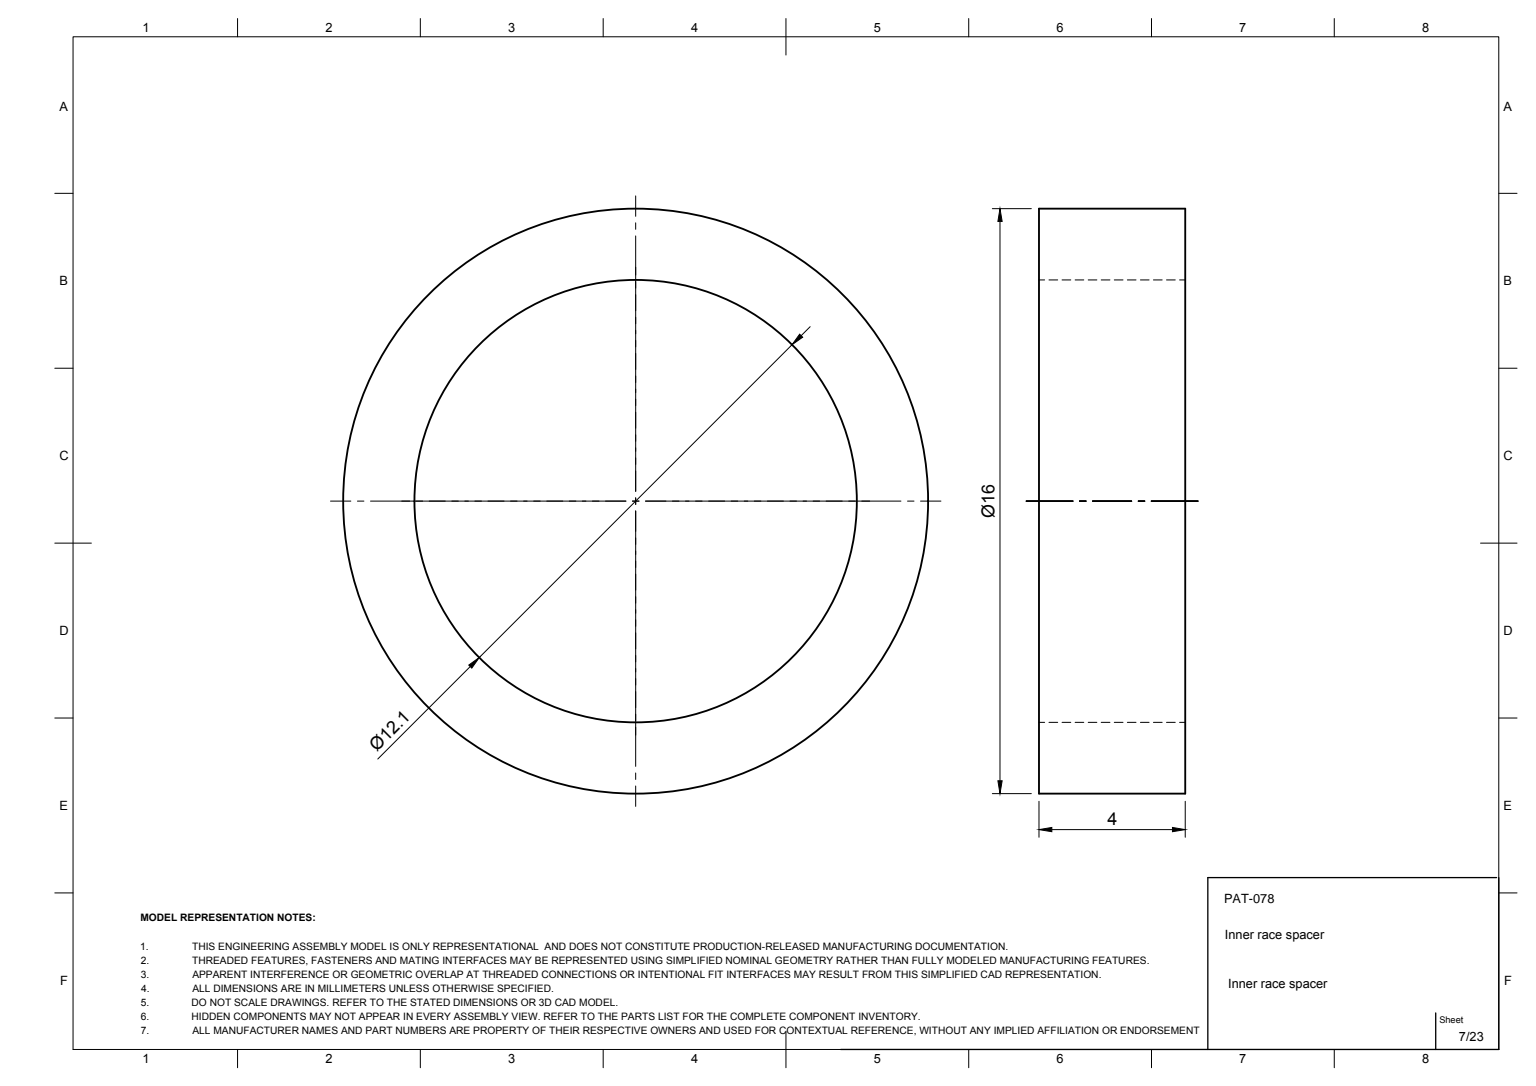
ISO-10303-21;
HEADER;
/* Generated by software containing ST-Developer
 * from STEP Tools, Inc. (www.steptools.com) 
 */

FILE_DESCRIPTION(
/* description */ ('Pedal-braked fixed caster'),
/* implementation_level */ '2;1');

FILE_NAME(
/* name */ 'Inner race spacer.step',
/* time_stamp */ '2026-10-28T03:26:52-07:00',
/* author */ (''),
/* organization */ (''),
/* preprocessor_version */ 'ST-DEVELOPER v20.2',
/* originating_system */ 'Autodesk Translation Framework v15.17.0.0',
/* authorisation */ '');

FILE_SCHEMA (('AUTOMOTIVE_DESIGN { 1 0 10303 214 3 1 1 }'));
ENDSEC;

DATA;
#10=MECHANICAL_DESIGN_GEOMETRIC_PRESENTATION_REPRESENTATION('',(#208),#5734);
#174=SHAPE_REPRESENTATION_RELATIONSHIP('SRR','None',#5812,#191);
#191=ADVANCED_BREP_SHAPE_REPRESENTATION('',(#232),#5716);
#208=STYLED_ITEM('',(#5984),#232);
#232=MANIFOLD_SOLID_BREP('Body1',#2989);
#264=CYLINDRICAL_SURFACE('',#3276,0.605);
#265=CYLINDRICAL_SURFACE('',#3279,0.8);
#313=FACE_BOUND('',#724,.T.);
#314=FACE_BOUND('',#726,.T.);
#362=CIRCLE('',#3277,0.605);
#363=CIRCLE('',#3278,0.605);
#364=CIRCLE('',#3280,0.8);
#365=CIRCLE('',#3281,0.8);
#525=FACE_OUTER_BOUND('',#721,.T.);
#526=FACE_OUTER_BOUND('',#722,.T.);
#527=FACE_OUTER_BOUND('',#723,.T.);
#528=FACE_OUTER_BOUND('',#725,.T.);
#721=EDGE_LOOP('',(#2186,#2187,#2188,#2189));
#722=EDGE_LOOP('',(#2190,#2191,#2192,#2193));
#723=EDGE_LOOP('',(#2194));
#724=EDGE_LOOP('',(#2195));
#725=EDGE_LOOP('',(#2196));
#726=EDGE_LOOP('',(#2197));
#978=LINE('',#4758,#1190);
#979=LINE('',#4764,#1191);
#1190=VECTOR('',#3818,0.605);
#1191=VECTOR('',#3825,0.8);
#1383=VERTEX_POINT('',#4755);
#1384=VERTEX_POINT('',#4757);
#1385=VERTEX_POINT('',#4761);
#1386=VERTEX_POINT('',#4763);
#1683=EDGE_CURVE('',#1383,#1383,#362,.T.);
#1684=EDGE_CURVE('',#1383,#1384,#978,.T.);
#1685=EDGE_CURVE('',#1384,#1384,#363,.T.);
#1686=EDGE_CURVE('',#1385,#1385,#364,.T.);
#1687=EDGE_CURVE('',#1385,#1386,#979,.T.);
#1688=EDGE_CURVE('',#1386,#1386,#365,.T.);
#2186=ORIENTED_EDGE('',*,*,#1683,.F.);
#2187=ORIENTED_EDGE('',*,*,#1684,.T.);
#2188=ORIENTED_EDGE('',*,*,#1685,.T.);
#2189=ORIENTED_EDGE('',*,*,#1684,.F.);
#2190=ORIENTED_EDGE('',*,*,#1686,.F.);
#2191=ORIENTED_EDGE('',*,*,#1687,.T.);
#2192=ORIENTED_EDGE('',*,*,#1688,.T.);
#2193=ORIENTED_EDGE('',*,*,#1687,.F.);
#2194=ORIENTED_EDGE('',*,*,#1686,.T.);
#2195=ORIENTED_EDGE('',*,*,#1683,.T.);
#2196=ORIENTED_EDGE('',*,*,#1688,.F.);
#2197=ORIENTED_EDGE('',*,*,#1685,.F.);
#2738=PLANE('',#3282);
#2739=PLANE('',#3283);
#2858=ADVANCED_FACE('',(#525),#264,.F.);
#2859=ADVANCED_FACE('',(#526),#265,.T.);
#2860=ADVANCED_FACE('',(#527,#313),#2738,.T.);
#2861=ADVANCED_FACE('',(#528,#314),#2739,.F.);
#2989=CLOSED_SHELL('',(#2858,#2859,#2860,#2861));
#3275=AXIS2_PLACEMENT_3D('',#4753,#3812,#3813);
#3276=AXIS2_PLACEMENT_3D('',#4754,#3814,#3815);
#3277=AXIS2_PLACEMENT_3D('',#4756,#3816,#3817);
#3278=AXIS2_PLACEMENT_3D('',#4759,#3819,#3820);
#3279=AXIS2_PLACEMENT_3D('',#4760,#3821,#3822);
#3280=AXIS2_PLACEMENT_3D('',#4762,#3823,#3824);
#3281=AXIS2_PLACEMENT_3D('',#4765,#3826,#3827);
#3282=AXIS2_PLACEMENT_3D('',#4766,#3828,#3829);
#3283=AXIS2_PLACEMENT_3D('',#4767,#3830,#3831);
#3812=DIRECTION('axis',(0.,0.,1.));
#3813=DIRECTION('refdir',(1.,0.,0.));
#3814=DIRECTION('center_axis',(0.,1.,0.));
#3815=DIRECTION('ref_axis',(1.,0.,0.));
#3816=DIRECTION('center_axis',(0.,-1.,0.));
#3817=DIRECTION('ref_axis',(1.,0.,0.));
#3818=DIRECTION('',(0.,-1.,0.));
#3819=DIRECTION('center_axis',(0.,-1.,0.));
#3820=DIRECTION('ref_axis',(1.,0.,0.));
#3821=DIRECTION('center_axis',(0.,1.,0.));
#3822=DIRECTION('ref_axis',(1.,0.,0.));
#3823=DIRECTION('center_axis',(0.,1.,0.));
#3824=DIRECTION('ref_axis',(1.,0.,0.));
#3825=DIRECTION('',(0.,-1.,0.));
#3826=DIRECTION('center_axis',(0.,1.,0.));
#3827=DIRECTION('ref_axis',(1.,0.,0.));
#3828=DIRECTION('center_axis',(0.,1.,0.));
#3829=DIRECTION('ref_axis',(1.,0.,0.));
#3830=DIRECTION('center_axis',(0.,1.,0.));
#3831=DIRECTION('ref_axis',(1.,0.,0.));
#4753=CARTESIAN_POINT('',(0.,0.,0.));
#4754=CARTESIAN_POINT('Origin',(0.,4.5,10.));
#4755=CARTESIAN_POINT('',(-0.605,4.9,10.));
#4756=CARTESIAN_POINT('Origin',(0.,4.9,10.));
#4757=CARTESIAN_POINT('',(-0.605,4.5,10.));
#4758=CARTESIAN_POINT('',(-0.605,4.5,10.));
#4759=CARTESIAN_POINT('Origin',(0.,4.5,10.));
#4760=CARTESIAN_POINT('Origin',(0.,4.5,10.));
#4761=CARTESIAN_POINT('',(-0.8,4.9,10.));
#4762=CARTESIAN_POINT('Origin',(0.,4.9,10.));
#4763=CARTESIAN_POINT('',(-0.8,4.5,10.));
#4764=CARTESIAN_POINT('',(-0.8,4.5,10.));
#4765=CARTESIAN_POINT('Origin',(0.,4.5,10.));
#4766=CARTESIAN_POINT('Origin',(0.,4.9,10.));
#4767=CARTESIAN_POINT('Origin',(0.,4.5,10.));
#5693=UNCERTAINTY_MEASURE_WITH_UNIT(LENGTH_MEASURE(0.001),#5735,
'DISTANCE_ACCURACY_VALUE',
'Maximum model space distance between geometric entities at asserted c
onnectivities');
#5711=UNCERTAINTY_MEASURE_WITH_UNIT(LENGTH_MEASURE(0.001),#5735,
'DISTANCE_ACCURACY_VALUE',
'Maximum model space distance between geometric entities at asserted c
onnectivities');
#5716=(
GEOMETRIC_REPRESENTATION_CONTEXT(3)
GLOBAL_UNCERTAINTY_ASSIGNED_CONTEXT((#5693))
GLOBAL_UNIT_ASSIGNED_CONTEXT((#5735,#5737,#5738))
REPRESENTATION_CONTEXT('','3D')
);
#5734=(
GEOMETRIC_REPRESENTATION_CONTEXT(3)
GLOBAL_UNCERTAINTY_ASSIGNED_CONTEXT((#5711))
GLOBAL_UNIT_ASSIGNED_CONTEXT((#5735,#5737,#5738))
REPRESENTATION_CONTEXT('','3D')
);
#5735=(
LENGTH_UNIT()
NAMED_UNIT(*)
SI_UNIT(.CENTI.,.METRE.)
);
#5737=(
NAMED_UNIT(*)
PLANE_ANGLE_UNIT()
SI_UNIT($,.RADIAN.)
);
#5738=(
NAMED_UNIT(*)
SI_UNIT($,.STERADIAN.)
SOLID_ANGLE_UNIT()
);
#5743=SHAPE_DEFINITION_REPRESENTATION(#5765,#5812);
#5765=PRODUCT_DEFINITION_SHAPE('',$,#5835);
#5812=SHAPE_REPRESENTATION('',(#3275),#5716);
#5830=PRODUCT_DEFINITION_CONTEXT('part definition',#5898,'design');
#5835=PRODUCT_DEFINITION('Inner race spacer','Inner race spacer',#5857,
#5830);
#5857=PRODUCT_DEFINITION_FORMATION('',$,#5904);
#5898=APPLICATION_CONTEXT(
'Core Data for Automotive Mechanical Design Process');
#5899=PRODUCT_CONTEXT('part definition',#5898,'mechanical');
#5904=PRODUCT('Inner race spacer','Inner race spacer',
'Inner race spacer',(#5899));
#5978=COLOUR_RGB('Grey',0.48,0.52,0.57);
#5979=FILL_AREA_STYLE_COLOUR('',#5978);
#5980=FILL_AREA_STYLE('',(#5979));
#5981=SURFACE_STYLE_FILL_AREA(#5980);
#5982=SURFACE_SIDE_STYLE('',(#5981));
#5983=SURFACE_STYLE_USAGE(.BOTH.,#5982);
#5984=PRESENTATION_STYLE_ASSIGNMENT((#5983));
ENDSEC;
END-ISO-10303-21;
